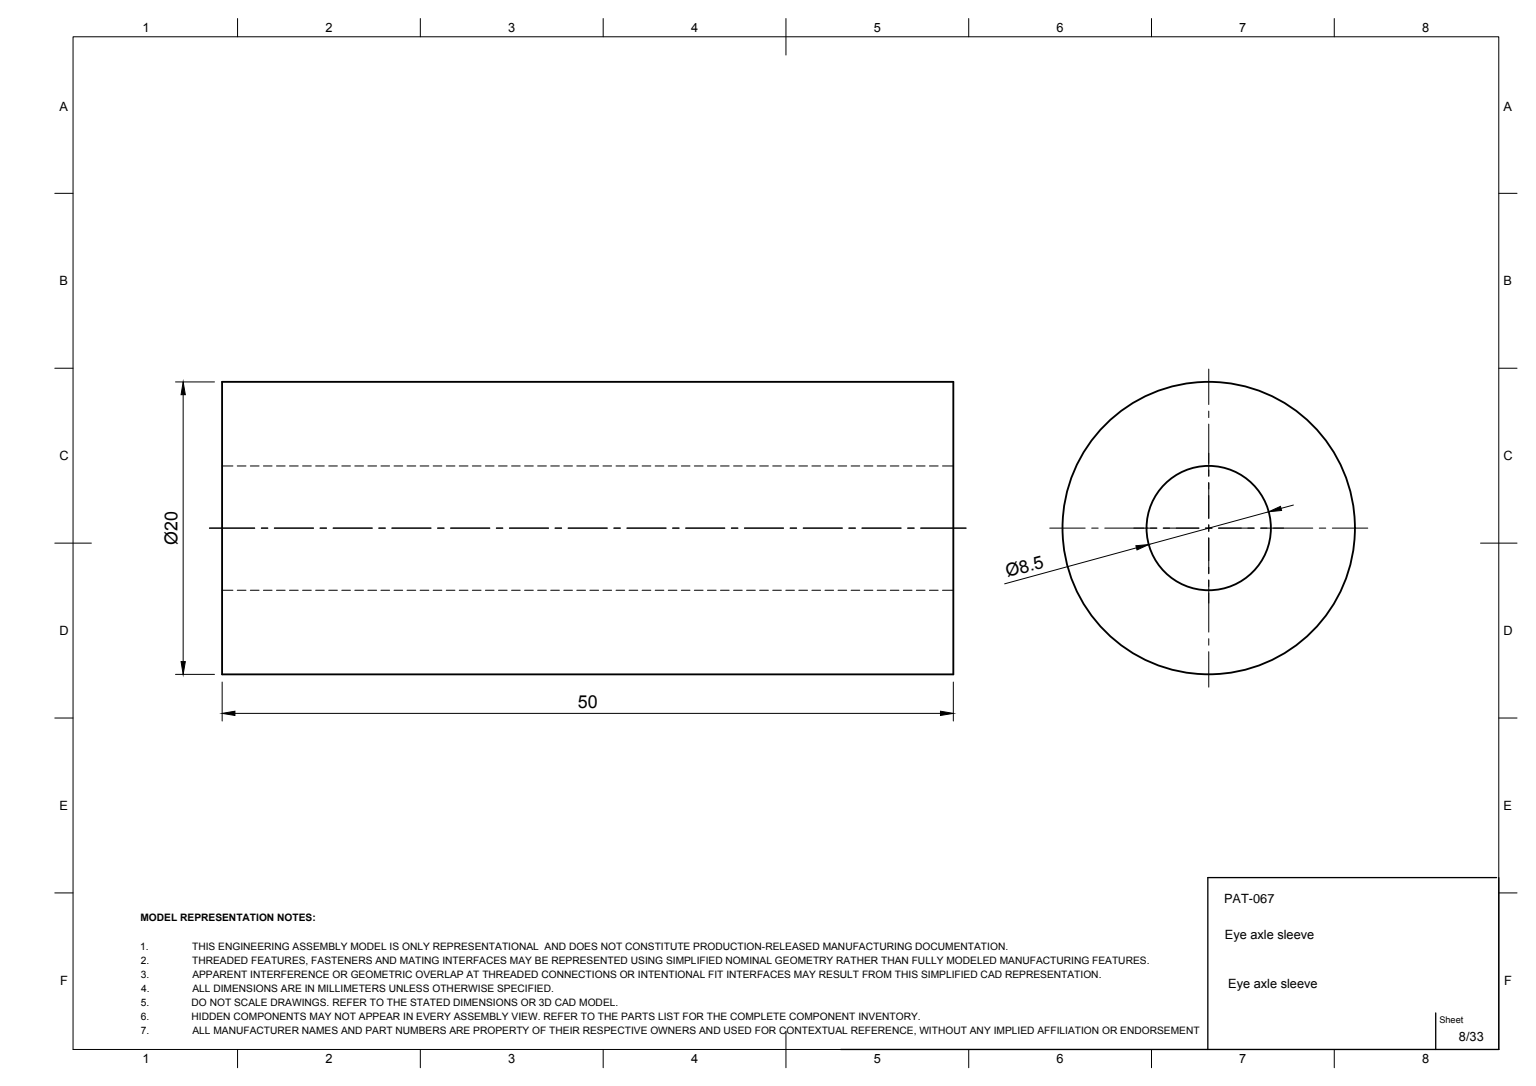
ISO-10303-21;
HEADER;
/* Generated by software containing ST-Developer
 * from STEP Tools, Inc. (www.steptools.com) 
 */

FILE_DESCRIPTION(
/* description */ ('Lifting hook block with sheave'),
/* implementation_level */ '2;1');

FILE_NAME(
/* name */ 'Eye axle sleeve.step',
/* time_stamp */ '2026-10-28T03:23:54-07:00',
/* author */ (''),
/* organization */ (''),
/* preprocessor_version */ 'ST-DEVELOPER v20.2',
/* originating_system */ 'Autodesk Translation Framework v15.17.0.0',
/* authorisation */ '');

FILE_SCHEMA (('AUTOMOTIVE_DESIGN { 1 0 10303 214 3 1 1 }'));
ENDSEC;

DATA;
#10=MECHANICAL_DESIGN_GEOMETRIC_PRESENTATION_REPRESENTATION('',(#354),#9391);
#294=SHAPE_REPRESENTATION_RELATIONSHIP('SRR','None',#9525,#324);
#324=ADVANCED_BREP_SHAPE_REPRESENTATION('',(#392),#9360);
#354=STYLED_ITEM('',(#9759),#392);
#392=MANIFOLD_SOLID_BREP('Body1',#4890);
#521=LINE('',#7911,#809);
#522=LINE('',#7917,#810);
#809=VECTOR('',#6308,0.425);
#810=VECTOR('',#6315,1.);
#1029=CYLINDRICAL_SURFACE('',#5398,0.425);
#1030=CYLINDRICAL_SURFACE('',#5401,1.);
#1141=FACE_BOUND('',#1607,.T.);
#1142=FACE_BOUND('',#1609,.T.);
#1281=FACE_OUTER_BOUND('',#1604,.T.);
#1282=FACE_OUTER_BOUND('',#1605,.T.);
#1283=FACE_OUTER_BOUND('',#1606,.T.);
#1284=FACE_OUTER_BOUND('',#1608,.T.);
#1604=EDGE_LOOP('',(#3572,#3573,#3574,#3575));
#1605=EDGE_LOOP('',(#3576,#3577,#3578,#3579));
#1606=EDGE_LOOP('',(#3580));
#1607=EDGE_LOOP('',(#3581));
#1608=EDGE_LOOP('',(#3582));
#1609=EDGE_LOOP('',(#3583));
#1989=CIRCLE('',#5399,0.425);
#1990=CIRCLE('',#5400,0.425);
#1991=CIRCLE('',#5402,1.);
#1992=CIRCLE('',#5403,1.);
#2322=VERTEX_POINT('',#7908);
#2323=VERTEX_POINT('',#7910);
#2324=VERTEX_POINT('',#7914);
#2325=VERTEX_POINT('',#7916);
#2790=EDGE_CURVE('',#2322,#2322,#1989,.T.);
#2791=EDGE_CURVE('',#2322,#2323,#521,.T.);
#2792=EDGE_CURVE('',#2323,#2323,#1990,.T.);
#2793=EDGE_CURVE('',#2324,#2324,#1991,.T.);
#2794=EDGE_CURVE('',#2324,#2325,#522,.T.);
#2795=EDGE_CURVE('',#2325,#2325,#1992,.T.);
#3572=ORIENTED_EDGE('',*,*,#2790,.F.);
#3573=ORIENTED_EDGE('',*,*,#2791,.T.);
#3574=ORIENTED_EDGE('',*,*,#2792,.T.);
#3575=ORIENTED_EDGE('',*,*,#2791,.F.);
#3576=ORIENTED_EDGE('',*,*,#2793,.F.);
#3577=ORIENTED_EDGE('',*,*,#2794,.T.);
#3578=ORIENTED_EDGE('',*,*,#2795,.T.);
#3579=ORIENTED_EDGE('',*,*,#2794,.F.);
#3580=ORIENTED_EDGE('',*,*,#2793,.T.);
#3581=ORIENTED_EDGE('',*,*,#2790,.T.);
#3582=ORIENTED_EDGE('',*,*,#2795,.F.);
#3583=ORIENTED_EDGE('',*,*,#2792,.F.);
#4482=PLANE('',#5404);
#4483=PLANE('',#5405);
#4657=ADVANCED_FACE('',(#1281),#1029,.F.);
#4658=ADVANCED_FACE('',(#1282),#1030,.T.);
#4659=ADVANCED_FACE('',(#1283,#1141),#4482,.T.);
#4660=ADVANCED_FACE('',(#1284,#1142),#4483,.F.);
#4890=CLOSED_SHELL('',(#4657,#4658,#4659,#4660));
#5397=AXIS2_PLACEMENT_3D('',#7906,#6302,#6303);
#5398=AXIS2_PLACEMENT_3D('',#7907,#6304,#6305);
#5399=AXIS2_PLACEMENT_3D('',#7909,#6306,#6307);
#5400=AXIS2_PLACEMENT_3D('',#7912,#6309,#6310);
#5401=AXIS2_PLACEMENT_3D('',#7913,#6311,#6312);
#5402=AXIS2_PLACEMENT_3D('',#7915,#6313,#6314);
#5403=AXIS2_PLACEMENT_3D('',#7918,#6316,#6317);
#5404=AXIS2_PLACEMENT_3D('',#7919,#6318,#6319);
#5405=AXIS2_PLACEMENT_3D('',#7920,#6320,#6321);
#6302=DIRECTION('axis',(0.,0.,1.));
#6303=DIRECTION('refdir',(1.,0.,0.));
#6304=DIRECTION('center_axis',(0.,1.,0.));
#6305=DIRECTION('ref_axis',(1.,0.,0.));
#6306=DIRECTION('center_axis',(0.,-1.,0.));
#6307=DIRECTION('ref_axis',(1.,0.,0.));
#6308=DIRECTION('',(0.,-1.,0.));
#6309=DIRECTION('center_axis',(0.,-1.,0.));
#6310=DIRECTION('ref_axis',(1.,0.,0.));
#6311=DIRECTION('center_axis',(0.,1.,0.));
#6312=DIRECTION('ref_axis',(1.,0.,0.));
#6313=DIRECTION('center_axis',(0.,1.,0.));
#6314=DIRECTION('ref_axis',(1.,0.,0.));
#6315=DIRECTION('',(0.,-1.,0.));
#6316=DIRECTION('center_axis',(0.,1.,0.));
#6317=DIRECTION('ref_axis',(1.,0.,0.));
#6318=DIRECTION('center_axis',(0.,1.,0.));
#6319=DIRECTION('ref_axis',(1.,0.,0.));
#6320=DIRECTION('center_axis',(0.,1.,0.));
#6321=DIRECTION('ref_axis',(1.,0.,0.));
#7906=CARTESIAN_POINT('',(0.,0.,0.));
#7907=CARTESIAN_POINT('Origin',(0.,-2.5,20.5));
#7908=CARTESIAN_POINT('',(-0.425,2.5,20.5));
#7909=CARTESIAN_POINT('Origin',(0.,2.5,20.5));
#7910=CARTESIAN_POINT('',(-0.425,-2.5,20.5));
#7911=CARTESIAN_POINT('',(-0.425,-2.5,20.5));
#7912=CARTESIAN_POINT('Origin',(0.,-2.5,20.5));
#7913=CARTESIAN_POINT('Origin',(0.,-2.5,20.5));
#7914=CARTESIAN_POINT('',(-1.,2.5,20.5));
#7915=CARTESIAN_POINT('Origin',(0.,2.5,20.5));
#7916=CARTESIAN_POINT('',(-1.,-2.5,20.5));
#7917=CARTESIAN_POINT('',(-1.,-2.5,20.5));
#7918=CARTESIAN_POINT('Origin',(0.,-2.5,20.5));
#7919=CARTESIAN_POINT('Origin',(0.,2.5,20.5));
#7920=CARTESIAN_POINT('Origin',(0.,-2.5,20.5));
#9323=UNCERTAINTY_MEASURE_WITH_UNIT(LENGTH_MEASURE(0.001),#9392,
'DISTANCE_ACCURACY_VALUE',
'Maximum model space distance between geometric entities at asserted c
onnectivities');
#9354=UNCERTAINTY_MEASURE_WITH_UNIT(LENGTH_MEASURE(0.001),#9392,
'DISTANCE_ACCURACY_VALUE',
'Maximum model space distance between geometric entities at asserted c
onnectivities');
#9360=(
GEOMETRIC_REPRESENTATION_CONTEXT(3)
GLOBAL_UNCERTAINTY_ASSIGNED_CONTEXT((#9323))
GLOBAL_UNIT_ASSIGNED_CONTEXT((#9392,#9394,#9395))
REPRESENTATION_CONTEXT('','3D')
);
#9391=(
GEOMETRIC_REPRESENTATION_CONTEXT(3)
GLOBAL_UNCERTAINTY_ASSIGNED_CONTEXT((#9354))
GLOBAL_UNIT_ASSIGNED_CONTEXT((#9392,#9394,#9395))
REPRESENTATION_CONTEXT('','3D')
);
#9392=(
LENGTH_UNIT()
NAMED_UNIT(*)
SI_UNIT(.CENTI.,.METRE.)
);
#9394=(
NAMED_UNIT(*)
PLANE_ANGLE_UNIT()
SI_UNIT($,.RADIAN.)
);
#9395=(
NAMED_UNIT(*)
SI_UNIT($,.STERADIAN.)
SOLID_ANGLE_UNIT()
);
#9401=SHAPE_DEFINITION_REPRESENTATION(#9437,#9525);
#9437=PRODUCT_DEFINITION_SHAPE('',$,#9562);
#9525=SHAPE_REPRESENTATION('',(#5397),#9360);
#9556=PRODUCT_DEFINITION_CONTEXT('part definition',#9666,'design');
#9562=PRODUCT_DEFINITION('Eye axle sleeve','Eye axle sleeve',#9598,#9556);
#9598=PRODUCT_DEFINITION_FORMATION('',$,#9673);
#9666=APPLICATION_CONTEXT(
'Core Data for Automotive Mechanical Design Process');
#9667=PRODUCT_CONTEXT('part definition',#9666,'mechanical');
#9673=PRODUCT('Eye axle sleeve','Eye axle sleeve','Eye axle sleeve',(#9667));
#9753=COLOUR_RGB('Grey',0.48,0.52,0.57);
#9754=FILL_AREA_STYLE_COLOUR('',#9753);
#9755=FILL_AREA_STYLE('',(#9754));
#9756=SURFACE_STYLE_FILL_AREA(#9755);
#9757=SURFACE_SIDE_STYLE('',(#9756));
#9758=SURFACE_STYLE_USAGE(.BOTH.,#9757);
#9759=PRESENTATION_STYLE_ASSIGNMENT((#9758));
ENDSEC;
END-ISO-10303-21;
